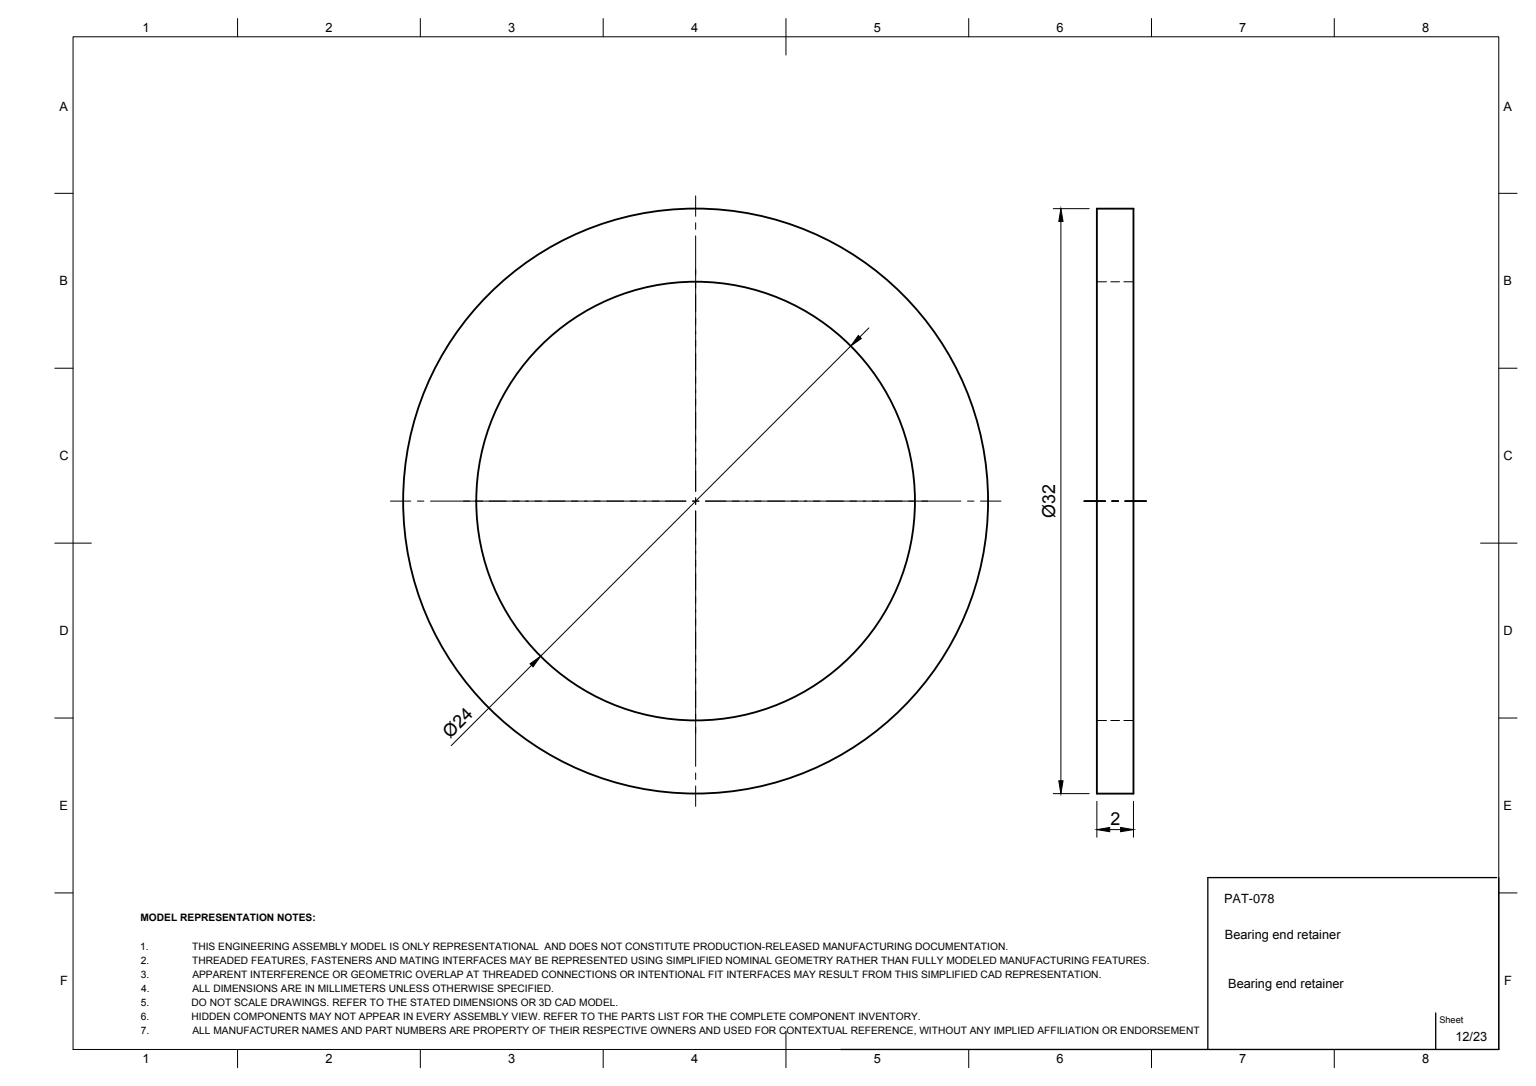
ISO-10303-21;
HEADER;
/* Generated by software containing ST-Developer
 * from STEP Tools, Inc. (www.steptools.com) 
 */

FILE_DESCRIPTION(
/* description */ ('Pedal-braked fixed caster'),
/* implementation_level */ '2;1');

FILE_NAME(
/* name */ 'Bearing end retainer.step',
/* time_stamp */ '2026-10-28T03:26:52-07:00',
/* author */ (''),
/* organization */ (''),
/* preprocessor_version */ 'ST-DEVELOPER v20.2',
/* originating_system */ 'Autodesk Translation Framework v15.17.0.0',
/* authorisation */ '');

FILE_SCHEMA (('AUTOMOTIVE_DESIGN { 1 0 10303 214 3 1 1 }'));
ENDSEC;

DATA;
#10=MECHANICAL_DESIGN_GEOMETRIC_PRESENTATION_REPRESENTATION('',(#227),#5734);
#186=SHAPE_REPRESENTATION_RELATIONSHIP('SRR','None',#5826,#203);
#203=ADVANCED_BREP_SHAPE_REPRESENTATION('',(#250),#5730);
#227=STYLED_ITEM('',(#5984),#250);
#250=MANIFOLD_SOLID_BREP('Body1',#3009);
#290=CYLINDRICAL_SURFACE('',#3516,1.2);
#291=CYLINDRICAL_SURFACE('',#3519,1.6);
#336=FACE_BOUND('',#854,.T.);
#337=FACE_BOUND('',#856,.T.);
#466=CIRCLE('',#3517,1.2);
#467=CIRCLE('',#3518,1.2);
#468=CIRCLE('',#3520,1.6);
#469=CIRCLE('',#3521,1.6);
#632=FACE_OUTER_BOUND('',#851,.T.);
#633=FACE_OUTER_BOUND('',#852,.T.);
#634=FACE_OUTER_BOUND('',#853,.T.);
#635=FACE_OUTER_BOUND('',#855,.T.);
#851=EDGE_LOOP('',(#2604,#2605,#2606,#2607));
#852=EDGE_LOOP('',(#2608,#2609,#2610,#2611));
#853=EDGE_LOOP('',(#2612));
#854=EDGE_LOOP('',(#2613));
#855=EDGE_LOOP('',(#2614));
#856=EDGE_LOOP('',(#2615));
#1051=LINE('',#5578,#1263);
#1052=LINE('',#5584,#1264);
#1263=VECTOR('',#4371,1.2);
#1264=VECTOR('',#4378,1.6);
#1528=VERTEX_POINT('',#5575);
#1529=VERTEX_POINT('',#5577);
#1530=VERTEX_POINT('',#5581);
#1531=VERTEX_POINT('',#5583);
#1892=EDGE_CURVE('',#1528,#1528,#466,.T.);
#1893=EDGE_CURVE('',#1528,#1529,#1051,.T.);
#1894=EDGE_CURVE('',#1529,#1529,#467,.T.);
#1895=EDGE_CURVE('',#1530,#1530,#468,.T.);
#1896=EDGE_CURVE('',#1530,#1531,#1052,.T.);
#1897=EDGE_CURVE('',#1531,#1531,#469,.T.);
#2604=ORIENTED_EDGE('',*,*,#1892,.F.);
#2605=ORIENTED_EDGE('',*,*,#1893,.T.);
#2606=ORIENTED_EDGE('',*,*,#1894,.T.);
#2607=ORIENTED_EDGE('',*,*,#1893,.F.);
#2608=ORIENTED_EDGE('',*,*,#1895,.F.);
#2609=ORIENTED_EDGE('',*,*,#1896,.T.);
#2610=ORIENTED_EDGE('',*,*,#1897,.T.);
#2611=ORIENTED_EDGE('',*,*,#1896,.F.);
#2612=ORIENTED_EDGE('',*,*,#1895,.T.);
#2613=ORIENTED_EDGE('',*,*,#1892,.T.);
#2614=ORIENTED_EDGE('',*,*,#1897,.F.);
#2615=ORIENTED_EDGE('',*,*,#1894,.F.);
#2792=PLANE('',#3522);
#2793=PLANE('',#3523);
#2965=ADVANCED_FACE('',(#632),#290,.F.);
#2966=ADVANCED_FACE('',(#633),#291,.T.);
#2967=ADVANCED_FACE('',(#634,#336),#2792,.T.);
#2968=ADVANCED_FACE('',(#635,#337),#2793,.F.);
#3009=CLOSED_SHELL('',(#2965,#2966,#2967,#2968));
#3515=AXIS2_PLACEMENT_3D('',#5573,#4365,#4366);
#3516=AXIS2_PLACEMENT_3D('',#5574,#4367,#4368);
#3517=AXIS2_PLACEMENT_3D('',#5576,#4369,#4370);
#3518=AXIS2_PLACEMENT_3D('',#5579,#4372,#4373);
#3519=AXIS2_PLACEMENT_3D('',#5580,#4374,#4375);
#3520=AXIS2_PLACEMENT_3D('',#5582,#4376,#4377);
#3521=AXIS2_PLACEMENT_3D('',#5585,#4379,#4380);
#3522=AXIS2_PLACEMENT_3D('',#5586,#4381,#4382);
#3523=AXIS2_PLACEMENT_3D('',#5587,#4383,#4384);
#4365=DIRECTION('axis',(0.,0.,1.));
#4366=DIRECTION('refdir',(1.,0.,0.));
#4367=DIRECTION('center_axis',(0.,1.,0.));
#4368=DIRECTION('ref_axis',(1.,0.,0.));
#4369=DIRECTION('center_axis',(0.,-1.,0.));
#4370=DIRECTION('ref_axis',(1.,0.,0.));
#4371=DIRECTION('',(0.,-1.,0.));
#4372=DIRECTION('center_axis',(0.,-1.,0.));
#4373=DIRECTION('ref_axis',(1.,0.,0.));
#4374=DIRECTION('center_axis',(0.,1.,0.));
#4375=DIRECTION('ref_axis',(1.,0.,0.));
#4376=DIRECTION('center_axis',(0.,1.,0.));
#4377=DIRECTION('ref_axis',(1.,0.,0.));
#4378=DIRECTION('',(0.,-1.,0.));
#4379=DIRECTION('center_axis',(0.,1.,0.));
#4380=DIRECTION('ref_axis',(1.,0.,0.));
#4381=DIRECTION('center_axis',(0.,1.,0.));
#4382=DIRECTION('ref_axis',(1.,0.,0.));
#4383=DIRECTION('center_axis',(0.,1.,0.));
#4384=DIRECTION('ref_axis',(1.,0.,0.));
#5573=CARTESIAN_POINT('',(0.,0.,0.));
#5574=CARTESIAN_POINT('Origin',(0.,1.1,3.5));
#5575=CARTESIAN_POINT('',(-1.2,1.3,3.5));
#5576=CARTESIAN_POINT('Origin',(0.,1.3,3.5));
#5577=CARTESIAN_POINT('',(-1.2,1.1,3.5));
#5578=CARTESIAN_POINT('',(-1.2,1.1,3.5));
#5579=CARTESIAN_POINT('Origin',(0.,1.1,3.5));
#5580=CARTESIAN_POINT('Origin',(0.,1.1,3.5));
#5581=CARTESIAN_POINT('',(-1.6,1.3,3.5));
#5582=CARTESIAN_POINT('Origin',(0.,1.3,3.5));
#5583=CARTESIAN_POINT('',(-1.6,1.1,3.5));
#5584=CARTESIAN_POINT('',(-1.6,1.1,3.5));
#5585=CARTESIAN_POINT('Origin',(0.,1.1,3.5));
#5586=CARTESIAN_POINT('Origin',(0.,1.3,3.5));
#5587=CARTESIAN_POINT('Origin',(0.,1.1,3.5));
#5707=UNCERTAINTY_MEASURE_WITH_UNIT(LENGTH_MEASURE(0.001),#5735,
'DISTANCE_ACCURACY_VALUE',
'Maximum model space distance between geometric entities at asserted c
onnectivities');
#5711=UNCERTAINTY_MEASURE_WITH_UNIT(LENGTH_MEASURE(0.001),#5735,
'DISTANCE_ACCURACY_VALUE',
'Maximum model space distance between geometric entities at asserted c
onnectivities');
#5730=(
GEOMETRIC_REPRESENTATION_CONTEXT(3)
GLOBAL_UNCERTAINTY_ASSIGNED_CONTEXT((#5707))
GLOBAL_UNIT_ASSIGNED_CONTEXT((#5735,#5737,#5738))
REPRESENTATION_CONTEXT('','3D')
);
#5734=(
GEOMETRIC_REPRESENTATION_CONTEXT(3)
GLOBAL_UNCERTAINTY_ASSIGNED_CONTEXT((#5711))
GLOBAL_UNIT_ASSIGNED_CONTEXT((#5735,#5737,#5738))
REPRESENTATION_CONTEXT('','3D')
);
#5735=(
LENGTH_UNIT()
NAMED_UNIT(*)
SI_UNIT(.CENTI.,.METRE.)
);
#5737=(
NAMED_UNIT(*)
PLANE_ANGLE_UNIT()
SI_UNIT($,.RADIAN.)
);
#5738=(
NAMED_UNIT(*)
SI_UNIT($,.STERADIAN.)
SOLID_ANGLE_UNIT()
);
#5757=SHAPE_DEFINITION_REPRESENTATION(#5794,#5826);
#5794=PRODUCT_DEFINITION_SHAPE('',$,#5849);
#5826=SHAPE_REPRESENTATION('',(#3515),#5730);
#5830=PRODUCT_DEFINITION_CONTEXT('part definition',#5898,'design');
#5849=PRODUCT_DEFINITION('Bearing end retainer','Bearing end retainer',
#5871,#5830);
#5871=PRODUCT_DEFINITION_FORMATION('',$,#5918);
#5898=APPLICATION_CONTEXT(
'Core Data for Automotive Mechanical Design Process');
#5899=PRODUCT_CONTEXT('part definition',#5898,'mechanical');
#5918=PRODUCT('Bearing end retainer','Bearing end retainer',
'Bearing end retainer',(#5899));
#5978=COLOUR_RGB('Grey',0.48,0.52,0.57);
#5979=FILL_AREA_STYLE_COLOUR('',#5978);
#5980=FILL_AREA_STYLE('',(#5979));
#5981=SURFACE_STYLE_FILL_AREA(#5980);
#5982=SURFACE_SIDE_STYLE('',(#5981));
#5983=SURFACE_STYLE_USAGE(.BOTH.,#5982);
#5984=PRESENTATION_STYLE_ASSIGNMENT((#5983));
ENDSEC;
END-ISO-10303-21;
